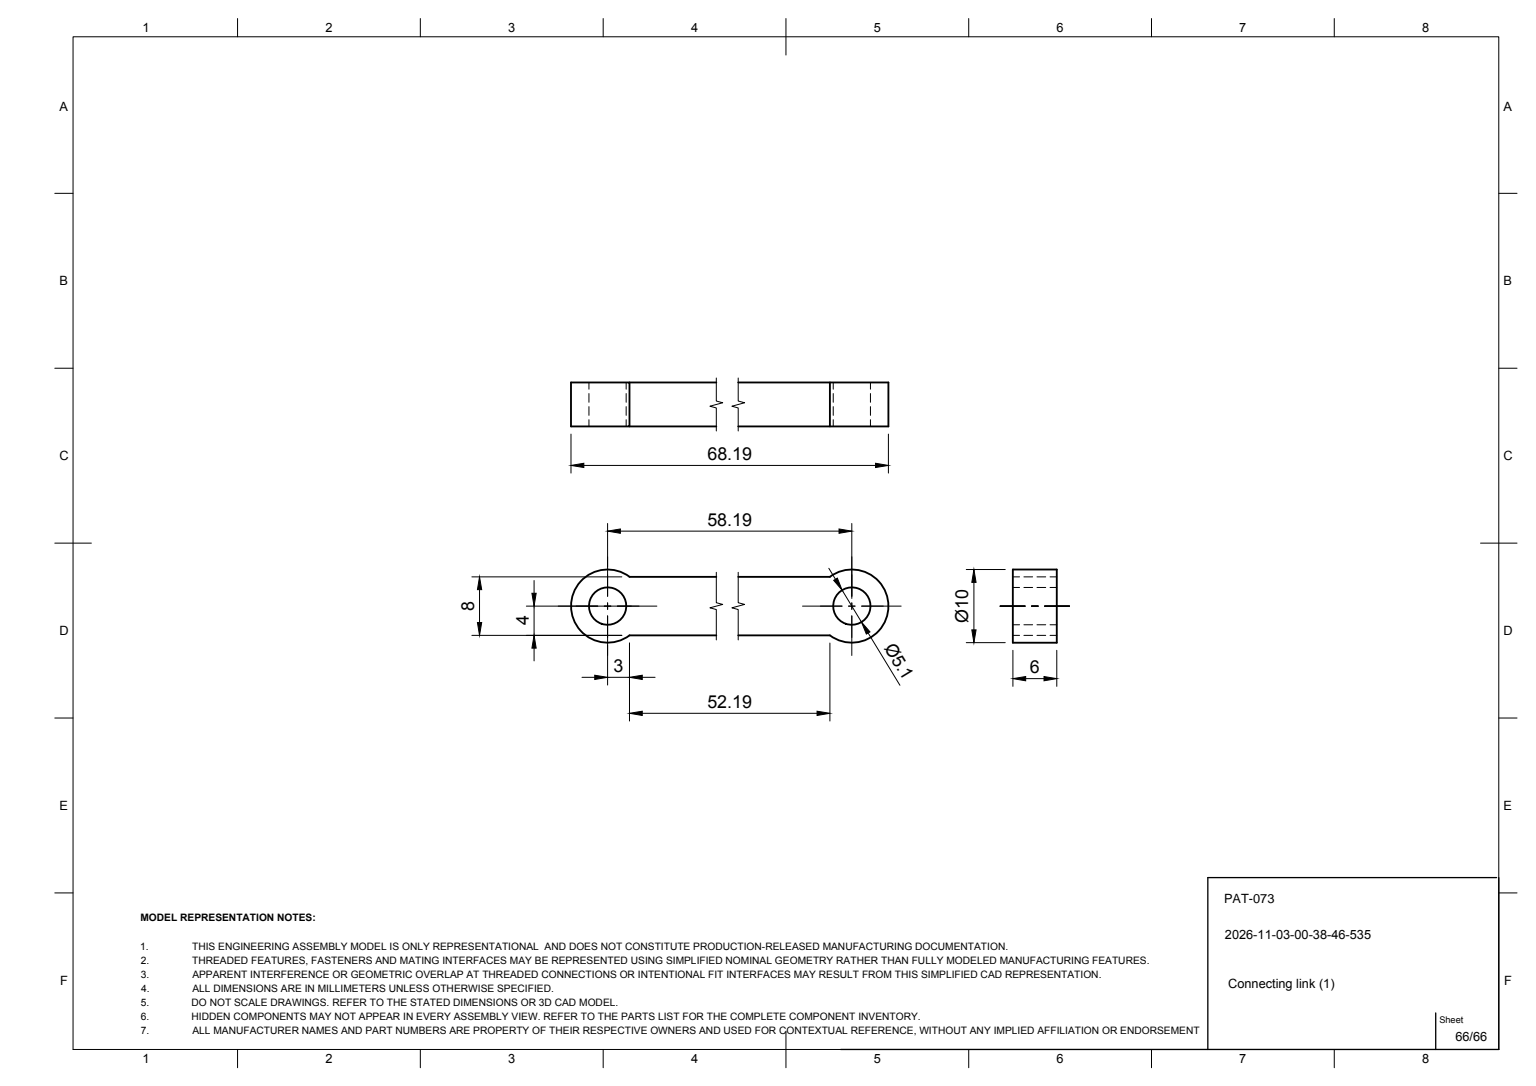
ISO-10303-21;
HEADER;
/* Generated by software containing ST-Developer
 * from STEP Tools, Inc. (www.steptools.com) 
 */

FILE_DESCRIPTION(
/* description */ ('Manual piston pump'),
/* implementation_level */ '2;1');

FILE_NAME(
/* name */ 'Connecting link (1).step',
/* time_stamp */ '2026-11-02T16:54:23-08:00',
/* author */ (''),
/* organization */ (''),
/* preprocessor_version */ 'ST-DEVELOPER v20.2',
/* originating_system */ 'Autodesk Translation Framework v15.17.0.0',
/* authorisation */ '');

FILE_SCHEMA (('AUTOMOTIVE_DESIGN { 1 0 10303 214 3 1 1 }'));
ENDSEC;

DATA;
#10=MECHANICAL_DESIGN_GEOMETRIC_PRESENTATION_REPRESENTATION('',(#759),#19043);
#624=SHAPE_REPRESENTATION_RELATIONSHIP('SRR','None',#19375,#687);
#687=ADVANCED_BREP_SHAPE_REPRESENTATION('',(#826),#19042);
#759=STYLED_ITEM('',(#19661),#826);
#826=MANIFOLD_SOLID_BREP('Body1',#9548);
#1044=FACE_BOUND('',#2655,.T.);
#1045=FACE_BOUND('',#2656,.T.);
#1046=FACE_BOUND('',#2661,.T.);
#1047=FACE_BOUND('',#2662,.T.);
#1288=CYLINDRICAL_SURFACE('',#11474,0.255000000000001);
#1289=CYLINDRICAL_SURFACE('',#11477,0.5);
#1290=CYLINDRICAL_SURFACE('',#11484,0.255);
#1291=CYLINDRICAL_SURFACE('',#11486,0.5);
#1859=FACE_OUTER_BOUND('',#2651,.T.);
#1860=FACE_OUTER_BOUND('',#2652,.T.);
#1861=FACE_OUTER_BOUND('',#2653,.T.);
#1862=FACE_OUTER_BOUND('',#2654,.T.);
#1863=FACE_OUTER_BOUND('',#2657,.T.);
#1864=FACE_OUTER_BOUND('',#2658,.T.);
#1865=FACE_OUTER_BOUND('',#2659,.T.);
#1866=FACE_OUTER_BOUND('',#2660,.T.);
#2651=EDGE_LOOP('',(#8537,#8538,#8539,#8540));
#2652=EDGE_LOOP('',(#8541,#8542,#8543,#8544));
#2653=EDGE_LOOP('',(#8545,#8546,#8547,#8548));
#2654=EDGE_LOOP('',(#8549,#8550,#8551,#8552));
#2655=EDGE_LOOP('',(#8553));
#2656=EDGE_LOOP('',(#8554));
#2657=EDGE_LOOP('',(#8555,#8556,#8557,#8558));
#2658=EDGE_LOOP('',(#8559,#8560,#8561,#8562));
#2659=EDGE_LOOP('',(#8563,#8564,#8565,#8566));
#2660=EDGE_LOOP('',(#8567,#8568,#8569,#8570));
#2661=EDGE_LOOP('',(#8571));
#2662=EDGE_LOOP('',(#8572));
#3139=CIRCLE('',#11475,0.255000000000001);
#3140=CIRCLE('',#11476,0.255000000000001);
#3141=CIRCLE('',#11478,0.5);
#3142=CIRCLE('',#11479,0.5);
#3143=CIRCLE('',#11482,0.5);
#3144=CIRCLE('',#11483,0.255);
#3145=CIRCLE('',#11485,0.255);
#3146=CIRCLE('',#11487,0.5);
#3741=LINE('',#18863,#4345);
#3742=LINE('',#18868,#4346);
#3743=LINE('',#18872,#4347);
#3744=LINE('',#18876,#4348);
#3745=LINE('',#18878,#4349);
#3746=LINE('',#18879,#4350);
#3747=LINE('',#18882,#4351);
#3748=LINE('',#18888,#4352);
#3749=LINE('',#18892,#4353);
#3750=LINE('',#18895,#4354);
#4345=VECTOR('',#14555,0.255000000000001);
#4346=VECTOR('',#14560,1.);
#4347=VECTOR('',#14563,1.);
#4348=VECTOR('',#14568,1.);
#4349=VECTOR('',#14569,1.);
#4350=VECTOR('',#14570,1.);
#4351=VECTOR('',#14573,1.);
#4352=VECTOR('',#14580,0.255);
#4353=VECTOR('',#14585,1.);
#4354=VECTOR('',#14590,1.);
#5111=VERTEX_POINT('',#18860);
#5112=VERTEX_POINT('',#18862);
#5113=VERTEX_POINT('',#18866);
#5114=VERTEX_POINT('',#18867);
#5115=VERTEX_POINT('',#18869);
#5116=VERTEX_POINT('',#18871);
#5117=VERTEX_POINT('',#18875);
#5118=VERTEX_POINT('',#18877);
#5119=VERTEX_POINT('',#18881);
#5120=VERTEX_POINT('',#18884);
#5121=VERTEX_POINT('',#18887);
#5122=VERTEX_POINT('',#18891);
#6255=EDGE_CURVE('',#5111,#5111,#3139,.T.);
#6256=EDGE_CURVE('',#5111,#5112,#3741,.T.);
#6257=EDGE_CURVE('',#5112,#5112,#3140,.T.);
#6258=EDGE_CURVE('',#5113,#5114,#3742,.T.);
#6259=EDGE_CURVE('',#5115,#5113,#3141,.T.);
#6260=EDGE_CURVE('',#5116,#5115,#3743,.T.);
#6261=EDGE_CURVE('',#5116,#5114,#3142,.T.);
#6262=EDGE_CURVE('',#5117,#5114,#3744,.T.);
#6263=EDGE_CURVE('',#5117,#5118,#3745,.T.);
#6264=EDGE_CURVE('',#5113,#5118,#3746,.T.);
#6265=EDGE_CURVE('',#5116,#5119,#3747,.T.);
#6266=EDGE_CURVE('',#5117,#5119,#3143,.T.);
#6267=EDGE_CURVE('',#5120,#5120,#3144,.T.);
#6268=EDGE_CURVE('',#5120,#5121,#3748,.T.);
#6269=EDGE_CURVE('',#5121,#5121,#3145,.T.);
#6270=EDGE_CURVE('',#5122,#5119,#3749,.T.);
#6271=EDGE_CURVE('',#5118,#5122,#3146,.T.);
#6272=EDGE_CURVE('',#5122,#5115,#3750,.T.);
#8537=ORIENTED_EDGE('',*,*,#6255,.F.);
#8538=ORIENTED_EDGE('',*,*,#6256,.T.);
#8539=ORIENTED_EDGE('',*,*,#6257,.F.);
#8540=ORIENTED_EDGE('',*,*,#6256,.F.);
#8541=ORIENTED_EDGE('',*,*,#6258,.F.);
#8542=ORIENTED_EDGE('',*,*,#6259,.F.);
#8543=ORIENTED_EDGE('',*,*,#6260,.F.);
#8544=ORIENTED_EDGE('',*,*,#6261,.T.);
#8545=ORIENTED_EDGE('',*,*,#6258,.T.);
#8546=ORIENTED_EDGE('',*,*,#6262,.F.);
#8547=ORIENTED_EDGE('',*,*,#6263,.T.);
#8548=ORIENTED_EDGE('',*,*,#6264,.F.);
#8549=ORIENTED_EDGE('',*,*,#6261,.F.);
#8550=ORIENTED_EDGE('',*,*,#6265,.T.);
#8551=ORIENTED_EDGE('',*,*,#6266,.F.);
#8552=ORIENTED_EDGE('',*,*,#6262,.T.);
#8553=ORIENTED_EDGE('',*,*,#6255,.T.);
#8554=ORIENTED_EDGE('',*,*,#6267,.T.);
#8555=ORIENTED_EDGE('',*,*,#6267,.F.);
#8556=ORIENTED_EDGE('',*,*,#6268,.T.);
#8557=ORIENTED_EDGE('',*,*,#6269,.F.);
#8558=ORIENTED_EDGE('',*,*,#6268,.F.);
#8559=ORIENTED_EDGE('',*,*,#6270,.F.);
#8560=ORIENTED_EDGE('',*,*,#6271,.F.);
#8561=ORIENTED_EDGE('',*,*,#6263,.F.);
#8562=ORIENTED_EDGE('',*,*,#6266,.T.);
#8563=ORIENTED_EDGE('',*,*,#6260,.T.);
#8564=ORIENTED_EDGE('',*,*,#6272,.F.);
#8565=ORIENTED_EDGE('',*,*,#6270,.T.);
#8566=ORIENTED_EDGE('',*,*,#6265,.F.);
#8567=ORIENTED_EDGE('',*,*,#6264,.T.);
#8568=ORIENTED_EDGE('',*,*,#6271,.T.);
#8569=ORIENTED_EDGE('',*,*,#6272,.T.);
#8570=ORIENTED_EDGE('',*,*,#6259,.T.);
#8571=ORIENTED_EDGE('',*,*,#6257,.T.);
#8572=ORIENTED_EDGE('',*,*,#6269,.T.);
#8893=PLANE('',#11480);
#8894=PLANE('',#11481);
#8895=PLANE('',#11488);
#8896=PLANE('',#11489);
#9464=ADVANCED_FACE('',(#1859),#1288,.F.);
#9465=ADVANCED_FACE('',(#1860),#1289,.T.);
#9466=ADVANCED_FACE('',(#1861),#8893,.T.);
#9467=ADVANCED_FACE('',(#1862,#1044,#1045),#8894,.F.);
#9468=ADVANCED_FACE('',(#1863),#1290,.F.);
#9469=ADVANCED_FACE('',(#1864),#1291,.T.);
#9470=ADVANCED_FACE('',(#1865),#8895,.T.);
#9471=ADVANCED_FACE('',(#1866,#1046,#1047),#8896,.T.);
#9548=CLOSED_SHELL('',(#9464,#9465,#9466,#9467,#9468,#9469,#9470,#9471));
#11473=AXIS2_PLACEMENT_3D('',#18858,#14549,#14550);
#11474=AXIS2_PLACEMENT_3D('',#18859,#14551,#14552);
#11475=AXIS2_PLACEMENT_3D('',#18861,#14553,#14554);
#11476=AXIS2_PLACEMENT_3D('',#18864,#14556,#14557);
#11477=AXIS2_PLACEMENT_3D('',#18865,#14558,#14559);
#11478=AXIS2_PLACEMENT_3D('',#18870,#14561,#14562);
#11479=AXIS2_PLACEMENT_3D('',#18873,#14564,#14565);
#11480=AXIS2_PLACEMENT_3D('',#18874,#14566,#14567);
#11481=AXIS2_PLACEMENT_3D('',#18880,#14571,#14572);
#11482=AXIS2_PLACEMENT_3D('',#18883,#14574,#14575);
#11483=AXIS2_PLACEMENT_3D('',#18885,#14576,#14577);
#11484=AXIS2_PLACEMENT_3D('',#18886,#14578,#14579);
#11485=AXIS2_PLACEMENT_3D('',#18889,#14581,#14582);
#11486=AXIS2_PLACEMENT_3D('',#18890,#14583,#14584);
#11487=AXIS2_PLACEMENT_3D('',#18893,#14586,#14587);
#11488=AXIS2_PLACEMENT_3D('',#18894,#14588,#14589);
#11489=AXIS2_PLACEMENT_3D('',#18896,#14591,#14592);
#14549=DIRECTION('axis',(0.,0.,1.));
#14550=DIRECTION('refdir',(1.,0.,0.));
#14551=DIRECTION('center_axis',(1.,0.,0.));
#14552=DIRECTION('ref_axis',(0.,0.,-1.));
#14553=DIRECTION('center_axis',(1.,0.,0.));
#14554=DIRECTION('ref_axis',(0.,0.,-1.));
#14555=DIRECTION('',(1.,0.,0.));
#14556=DIRECTION('center_axis',(-1.,0.,0.));
#14557=DIRECTION('ref_axis',(0.,0.,-1.));
#14558=DIRECTION('center_axis',(1.,0.,0.));
#14559=DIRECTION('ref_axis',(0.,-0.326520252798045,0.945190205468032));
#14560=DIRECTION('',(-1.,0.,0.));
#14561=DIRECTION('center_axis',(1.,0.,0.));
#14562=DIRECTION('ref_axis',(0.,0.,-1.));
#14563=DIRECTION('',(1.,0.,0.));
#14564=DIRECTION('center_axis',(1.,0.,0.));
#14565=DIRECTION('ref_axis',(0.,0.,-1.));
#14566=DIRECTION('center_axis',(0.,-0.945190205468031,-0.326520252798047));
#14567=DIRECTION('ref_axis',(0.,0.326520252798047,-0.945190205468031));
#14568=DIRECTION('',(0.,-0.326520252798047,0.945190205468031));
#14569=DIRECTION('',(1.,0.,0.));
#14570=DIRECTION('',(0.,0.326520252798047,-0.945190205468031));
#14571=DIRECTION('center_axis',(1.,0.,0.));
#14572=DIRECTION('ref_axis',(0.,0.,-1.));
#14573=DIRECTION('',(0.,0.326520252798047,-0.945190205468031));
#14574=DIRECTION('center_axis',(1.,0.,0.));
#14575=DIRECTION('ref_axis',(0.,0.,-1.));
#14576=DIRECTION('center_axis',(1.,0.,0.));
#14577=DIRECTION('ref_axis',(0.,0.,-1.));
#14578=DIRECTION('center_axis',(1.,0.,0.));
#14579=DIRECTION('ref_axis',(0.,0.,-1.));
#14580=DIRECTION('',(1.,0.,0.));
#14581=DIRECTION('center_axis',(-1.,0.,0.));
#14582=DIRECTION('ref_axis',(0.,0.,-1.));
#14583=DIRECTION('center_axis',(1.,0.,0.));
#14584=DIRECTION('ref_axis',(0.,0.,-1.));
#14585=DIRECTION('',(-1.,0.,0.));
#14586=DIRECTION('center_axis',(1.,0.,0.));
#14587=DIRECTION('ref_axis',(0.,0.,-1.));
#14588=DIRECTION('center_axis',(0.,0.945190205468031,0.326520252798047));
#14589=DIRECTION('ref_axis',(0.,-0.326520252798047,0.945190205468031));
#14590=DIRECTION('',(0.,-0.326520252798047,0.945190205468031));
#14591=DIRECTION('center_axis',(1.,0.,0.));
#14592=DIRECTION('ref_axis',(0.,0.,-1.));
#18858=CARTESIAN_POINT('',(0.,0.,0.));
#18859=CARTESIAN_POINT('Origin',(-0.4,-8.,10.));
#18860=CARTESIAN_POINT('',(-0.3,-8.,10.255));
#18861=CARTESIAN_POINT('Origin',(-0.3,-8.,10.));
#18862=CARTESIAN_POINT('',(0.3,-8.,10.255));
#18863=CARTESIAN_POINT('',(-0.4,-8.,10.255));
#18864=CARTESIAN_POINT('Origin',(0.3,-8.,10.));
#18865=CARTESIAN_POINT('Origin',(-0.3,-8.,10.));
#18866=CARTESIAN_POINT('',(0.3,-8.2801200063478,9.58583483724037));
#18867=CARTESIAN_POINT('',(-0.3,-8.2801200063478,9.58583483724037));
#18868=CARTESIAN_POINT('',(-0.3,-8.2801200063478,9.58583483724037));
#18869=CARTESIAN_POINT('',(0.3,-7.52396784197337,9.84705103947881));
#18870=CARTESIAN_POINT('Origin',(0.3,-8.,10.));
#18871=CARTESIAN_POINT('',(-0.3,-7.52396784197337,9.84705103947881));
#18872=CARTESIAN_POINT('',(-0.3,-7.52396784197337,9.84705103947881));
#18873=CARTESIAN_POINT('Origin',(-0.3,-8.,10.));
#18874=CARTESIAN_POINT('Origin',(-0.3,-8.37807608218721,9.86939189888078));
#18875=CARTESIAN_POINT('',(-0.3,-6.57603215802663,4.65294896052119));
#18876=CARTESIAN_POINT('',(-0.3,-6.47807608218721,4.36939189888078));
#18877=CARTESIAN_POINT('',(0.3,-6.57603215802663,4.65294896052119));
#18878=CARTESIAN_POINT('',(-0.3,-6.57603215802663,4.65294896052119));
#18879=CARTESIAN_POINT('',(0.3,-6.47807608218721,4.36939189888078));
#18880=CARTESIAN_POINT('Origin',(-0.3,-7.05,7.25));
#18881=CARTESIAN_POINT('',(-0.3,-5.8198799936522,4.91416516275963));
#18882=CARTESIAN_POINT('',(-0.3,-7.62192391781279,10.1306081011192));
#18883=CARTESIAN_POINT('Origin',(-0.3,-6.1,4.5));
#18884=CARTESIAN_POINT('',(-0.3,-6.1,4.755));
#18885=CARTESIAN_POINT('Origin',(-0.3,-6.1,4.5));
#18886=CARTESIAN_POINT('Origin',(-0.4,-6.1,4.5));
#18887=CARTESIAN_POINT('',(0.3,-6.1,4.755));
#18888=CARTESIAN_POINT('',(-0.4,-6.1,4.755));
#18889=CARTESIAN_POINT('Origin',(0.3,-6.1,4.5));
#18890=CARTESIAN_POINT('Origin',(-0.3,-6.1,4.5));
#18891=CARTESIAN_POINT('',(0.3,-5.8198799936522,4.91416516275963));
#18892=CARTESIAN_POINT('',(-0.3,-5.8198799936522,4.91416516275963));
#18893=CARTESIAN_POINT('Origin',(0.3,-6.1,4.5));
#18894=CARTESIAN_POINT('Origin',(-0.3,-5.72192391781279,4.63060810111922));
#18895=CARTESIAN_POINT('',(0.3,-7.62192391781279,10.1306081011192));
#18896=CARTESIAN_POINT('Origin',(0.3,-7.05,7.25));
#18971=UNCERTAINTY_MEASURE_WITH_UNIT(LENGTH_MEASURE(0.001),#19044,
'DISTANCE_ACCURACY_VALUE',
'Maximum model space distance between geometric entities at asserted c
onnectivities');
#18972=UNCERTAINTY_MEASURE_WITH_UNIT(LENGTH_MEASURE(0.001),#19044,
'DISTANCE_ACCURACY_VALUE',
'Maximum model space distance between geometric entities at asserted c
onnectivities');
#19042=(
GEOMETRIC_REPRESENTATION_CONTEXT(3)
GLOBAL_UNCERTAINTY_ASSIGNED_CONTEXT((#18971))
GLOBAL_UNIT_ASSIGNED_CONTEXT((#19044,#19046,#19047))
REPRESENTATION_CONTEXT('','3D')
);
#19043=(
GEOMETRIC_REPRESENTATION_CONTEXT(3)
GLOBAL_UNCERTAINTY_ASSIGNED_CONTEXT((#18972))
GLOBAL_UNIT_ASSIGNED_CONTEXT((#19044,#19046,#19047))
REPRESENTATION_CONTEXT('','3D')
);
#19044=(
LENGTH_UNIT()
NAMED_UNIT(*)
SI_UNIT(.CENTI.,.METRE.)
);
#19046=(
NAMED_UNIT(*)
PLANE_ANGLE_UNIT()
SI_UNIT($,.RADIAN.)
);
#19047=(
NAMED_UNIT(*)
SI_UNIT($,.STERADIAN.)
SOLID_ANGLE_UNIT()
);
#19117=SHAPE_DEFINITION_REPRESENTATION(#19300,#19375);
#19300=PRODUCT_DEFINITION_SHAPE('',$,#19446);
#19375=SHAPE_REPRESENTATION('',(#11473),#19042);
#19376=PRODUCT_DEFINITION_CONTEXT('part definition',#19588,'design');
#19446=PRODUCT_DEFINITION('2026-11-03-00-38-46-535',
'Connecting link (1)',#19516,#19376);
#19516=PRODUCT_DEFINITION_FORMATION('',$,#19659);
#19588=APPLICATION_CONTEXT(
'Core Data for Automotive Mechanical Design Process');
#19589=PRODUCT_CONTEXT('part definition',#19588,'mechanical');
#19659=PRODUCT('2026-11-03-00-38-46-535','Connecting link (1)',
'Connecting link',(#19589));
#19661=PRESENTATION_STYLE_ASSIGNMENT((#19667));
#19667=SURFACE_STYLE_USAGE(.BOTH.,#19673);
#19673=SURFACE_SIDE_STYLE('',(#19679));
#19679=SURFACE_STYLE_FILL_AREA(#19685);
#19685=FILL_AREA_STYLE('CAD Library Painted - Engineering blue',(#19691));
#19691=FILL_AREA_STYLE_COLOUR('CAD Library Painted - Engineering blue',
#19697);
#19697=COLOUR_RGB('CAD Library Painted - Engineering blue',0.12156862745098,
0.356862745098039,0.6);
ENDSEC;
END-ISO-10303-21;
